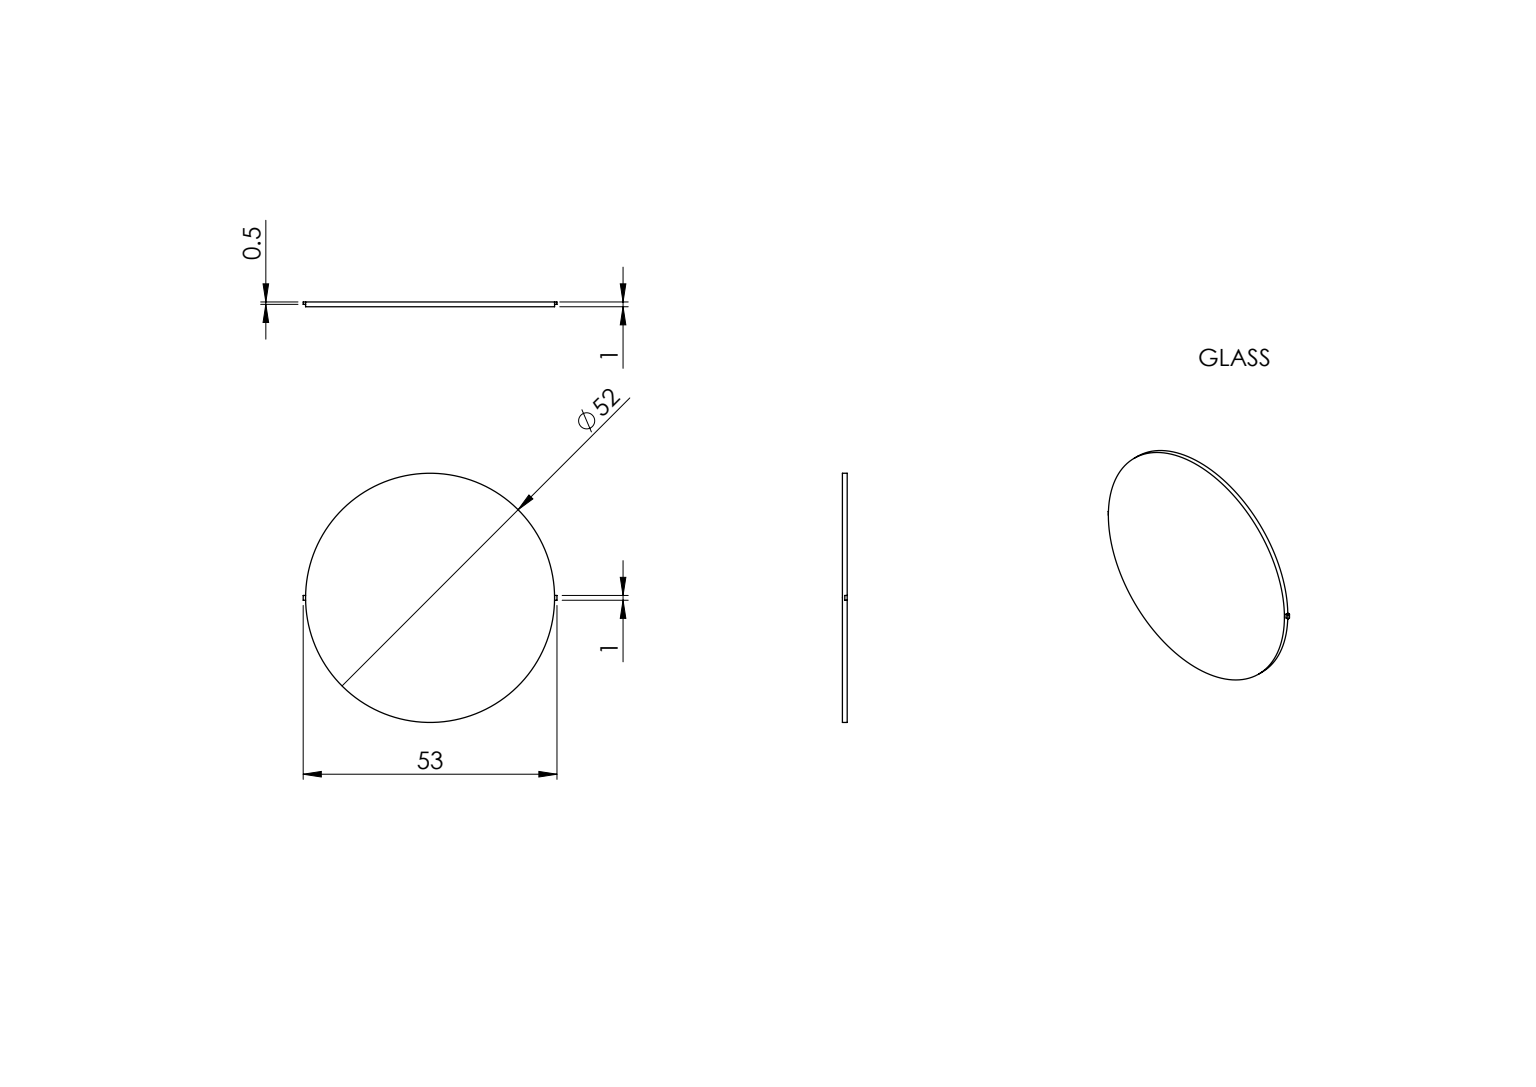
ISO-10303-21;
HEADER;
FILE_DESCRIPTION (('STEP AP214'),
    '1' );
FILE_NAME ('glass.step',
    '2026-10-26T11:20:31',
    ( '' ),
    ( '' ),
    'SwSTEP 2.0',
    'SolidWorks 2026',
    '' );
FILE_SCHEMA (( 'AUTOMOTIVE_DESIGN' ));
ENDSEC;

DATA;
#34=ORIENTED_EDGE ( 'NONE', *, *, #3765, .T. ) ;
#67=FACE_OUTER_BOUND ( 'NONE', #3163, .T. ) ;
#75=ORIENTED_EDGE ( 'NONE', *, *, #1897, .F. ) ;
#83=PLANE ( 'NONE',  #429 ) ;
#102=VERTEX_POINT ( 'NONE', #652 ) ;
#124=ORIENTED_EDGE ( 'NONE', *, *, #3765, .F. ) ;
#132=EDGE_CURVE ( 'NONE', #2734, #2850, #1760, .T. ) ;
#136=AXIS2_PLACEMENT_3D ( 'NONE', #3423, #167, #2705 ) ;
#142=EDGE_CURVE ( 'NONE', #3182, #1602, #2491, .T. ) ;
#147=CARTESIAN_POINT ( 'NONE',  ( 0.000000000000000000, 0.000000000000000000, 20.00000000000000000 ) ) ;
#167=DIRECTION ( 'NONE',  ( 0.000000000000000000, -0.000000000000000000, 1.000000000000000000 ) ) ;
#206=PRODUCT ( 'glass', 'glass', '', ( #2572 ) ) ;
#214=ORIENTED_EDGE ( 'NONE', *, *, #364, .F. ) ;
#229=EDGE_CURVE ( 'NONE', #3297, #3886, #3090, .T. ) ;
#234=CARTESIAN_POINT ( 'NONE',  ( 26.49999999999999645, -0.5000000000000000000, 19.50000000000000000 ) ) ;
#248=VECTOR ( 'NONE', #2476, 1000.000000000000000 ) ;
#285=LINE ( 'NONE', #1756, #509 ) ;
#331=PLANE ( 'NONE',  #3572 ) ;
#364=EDGE_CURVE ( 'NONE', #2850, #4511, #2465, .T. ) ;
#369=DIRECTION ( 'NONE',  ( -1.000000000000000000, 0.000000000000000000, 0.000000000000000000 ) ) ;
#389=CARTESIAN_POINT ( 'NONE',  ( 26.00000000000000711, 3.184081677783118980E-15, 20.00000000000000000 ) ) ;
#398=FACE_OUTER_BOUND ( 'NONE', #695, .T. ) ;
#413=VECTOR ( 'NONE', #4600, 1000.000000000000000 ) ;
#418=VERTEX_POINT ( 'NONE', #4346 ) ;
#422=APPLICATION_CONTEXT ( 'automotive_design' ) ;
#425=ADVANCED_FACE ( 'NONE', ( #2551 ), #3201, .T. ) ;
#426=ORIENTED_EDGE ( 'NONE', *, *, #1762, .F. ) ;
#429=AXIS2_PLACEMENT_3D ( 'NONE', #1371, #641, #2955 ) ;
#437=AXIS2_PLACEMENT_3D ( 'NONE', #3171, #2146, #3524 ) ;
#440=VECTOR ( 'NONE', #3448, 1000.000000000000000 ) ;
#456=VECTOR ( 'NONE', #3934, 1000.000000000000000 ) ;
#463=VECTOR ( 'NONE', #1245, 1000.000000000000000 ) ;
#483=ORIENTED_EDGE ( 'NONE', *, *, #4706, .T. ) ;
#488=CIRCLE ( 'NONE', #2609, 26.00000000000000711 ) ;
#492=ORIENTED_EDGE ( 'NONE', *, *, #132, .T. ) ;
#509=VECTOR ( 'NONE', #2115, 1000.000000000000000 ) ;
#517=CARTESIAN_POINT ( 'NONE',  ( 26.49999999999999645, 0.5000000000000000000, 19.00000000000000000 ) ) ;
#552=LINE ( 'NONE', #1733, #440 ) ;
#572=ORIENTED_EDGE ( 'NONE', *, *, #4588, .T. ) ;
#612=CARTESIAN_POINT ( 'NONE',  ( -25.99519186311192342, -0.5000000000000000000, 19.50000000000000000 ) ) ;
#620=ADVANCED_FACE ( 'NONE', ( #67 ), #1945, .T. ) ;
#625=CARTESIAN_POINT ( 'NONE',  ( 25.99519186311192342, -0.5000000000000000000, 19.50000000000000000 ) ) ;
#627=( NAMED_UNIT ( * ) SI_UNIT ( $, .STERADIAN. ) SOLID_ANGLE_UNIT ( ) );
#633=CARTESIAN_POINT ( 'NONE',  ( 26.49999999999999645, 0.5000000000000000000, 19.00000000000000000 ) ) ;
#641=DIRECTION ( 'NONE',  ( -1.000000000000000000, 0.000000000000000000, 0.000000000000000000 ) ) ;
#645=ORIENTED_EDGE ( 'NONE', *, *, #2272, .F. ) ;
#652=CARTESIAN_POINT ( 'NONE',  ( 26.49999999999999645, 0.5000000000000000000, 19.50000000000000000 ) ) ;
#672=FILL_AREA_STYLE ('',( #2807 ) ) ;
#676=DIRECTION ( 'NONE',  ( 1.000000000000000000, 0.000000000000000000, 0.000000000000000000 ) ) ;
#682=AXIS2_PLACEMENT_3D ( 'NONE', #4584, #4229, #972 ) ;
#695=EDGE_LOOP ( 'NONE', ( #214, #1153, #2156, #1634, #75 ) ) ;
#754=STYLED_ITEM('',(#4729),#2889);
#777=EDGE_CURVE ( 'NONE', #1588, #3297, #4191, .T. ) ;
#824=VECTOR ( 'NONE', #4005, 1000.000000000000000 ) ;
#827=ORIENTED_EDGE ( 'NONE', *, *, #3495, .T. ) ;
#835=ORIENTED_EDGE ( 'NONE', *, *, #777, .T. ) ;
#839=PRODUCT_DEFINITION ( 'UNKNOWN', '', #2243, #1713 ) ;
#856=ORIENTED_EDGE ( 'NONE', *, *, #4405, .T. ) ;
#863=EDGE_CURVE ( 'NONE', #4361, #4498, #4302, .T. ) ;
#888=DIRECTION ( 'NONE',  ( 1.000000000000000000, -0.000000000000000000, -0.000000000000000000 ) ) ;
#896=ADVANCED_FACE ( 'NONE', ( #1497 ), #83, .T. ) ;
#901=CARTESIAN_POINT ( 'NONE',  ( 0.000000000000000000, 0.000000000000000000, 19.50000000000000000 ) ) ;
#931=EDGE_LOOP ( 'NONE', ( #3447, #2373, #34, #4420, #3973, #4198, #492, #4425 ) ) ;
#935=ORIENTED_EDGE ( 'NONE', *, *, #2783, .T. ) ;
#960=ADVANCED_FACE ( 'NONE', ( #4674 ), #2853, .T. ) ;
#972=DIRECTION ( 'NONE',  ( 1.000000000000000000, 0.000000000000000000, 0.000000000000000000 ) ) ;
#981=ORIENTED_EDGE ( 'NONE', *, *, #1897, .T. ) ;
#983=LINE ( 'NONE', #4201, #2873 ) ;
#996=LINE ( 'NONE', #2062, #248 ) ;
#998=CARTESIAN_POINT ( 'NONE',  ( 26.49999999999999645, -0.5000000000000000000, 19.00000000000000000 ) ) ;
#1003=PRESENTATION_STYLE_ASSIGNMENT (( #2485 ) ) ;
#1010=ORIENTED_EDGE ( 'NONE', *, *, #142, .F. ) ;
#1029=CARTESIAN_POINT ( 'NONE',  ( 25.99519186311192342, -0.5000000000000000000, 20.00000000000000000 ) ) ;
#1037=COLOUR_RGB ( '',0.8941176470588234615, 0.8941176470588234615, 0.8941176470588234615 ) ;
#1039=CARTESIAN_POINT ( 'NONE',  ( -26.50000000000000355, 0.5000000000000000000, 19.50000000000000000 ) ) ;
#1045=CARTESIAN_POINT ( 'NONE',  ( 0.000000000000000000, 0.000000000000000000, 20.00000000000000000 ) ) ;
#1091=ADVANCED_FACE ( 'NONE', ( #398 ), #331, .T. ) ;
#1113=DIRECTION ( 'NONE',  ( 1.000000000000000000, 0.000000000000000000, 0.000000000000000000 ) ) ;
#1114=CYLINDRICAL_SURFACE ( 'NONE', #4514, 26.00000000000000711 ) ;
#1115=DIRECTION ( 'NONE',  ( 0.000000000000000000, 0.000000000000000000, -1.000000000000000000 ) ) ;
#1131=EDGE_CURVE ( 'NONE', #3723, #2120, #2345, .T. ) ;
#1138=CARTESIAN_POINT ( 'NONE',  ( 0.000000000000000000, 0.000000000000000000, 19.00000000000000000 ) ) ;
#1153=ORIENTED_EDGE ( 'NONE', *, *, #2783, .F. ) ;
#1184=( GEOMETRIC_REPRESENTATION_CONTEXT ( 3 ) GLOBAL_UNCERTAINTY_ASSIGNED_CONTEXT ( ( #1246 ) ) GLOBAL_UNIT_ASSIGNED_CONTEXT ( ( #1619, #2368, #2391 ) ) REPRESENTATION_CONTEXT ( 'NONE', 'WORKASPACE' ) );
#1218=ORIENTED_EDGE ( 'NONE', *, *, #4706, .F. ) ;
#1236=VECTOR ( 'NONE', #2396, 1000.000000000000000 ) ;
#1245=DIRECTION ( 'NONE',  ( 1.000000000000000000, -0.000000000000000000, -0.000000000000000000 ) ) ;
#1246=UNCERTAINTY_MEASURE_WITH_UNIT (LENGTH_MEASURE( 1.000000000000000082E-05 ), #1619, 'distance_accuracy_value', 'NONE');
#1249=EDGE_CURVE ( 'NONE', #3723, #4511, #4529, .T. ) ;
#1250=EDGE_CURVE ( 'NONE', #418, #102, #3047, .T. ) ;
#1289=ORIENTED_EDGE ( 'NONE', *, *, #4086, .T. ) ;
#1310=CARTESIAN_POINT ( 'NONE',  ( 0.000000000000000000, 0.000000000000000000, 19.50000000000000000 ) ) ;
#1332=CARTESIAN_POINT ( 'NONE',  ( 26.49999999999999645, -0.5000000000000000000, 19.50000000000000000 ) ) ;
#1346=CARTESIAN_POINT ( 'NONE',  ( 25.99519186311192342, 0.5000000000000000000, 20.00000000000000000 ) ) ;
#1350=ORIENTED_EDGE ( 'NONE', *, *, #4588, .F. ) ;
#1361=ADVANCED_FACE ( 'NONE', ( #3429 ), #3142, .F. ) ;
#1366=CARTESIAN_POINT ( 'NONE',  ( 26.49999999999999645, -0.5000000000000000000, 19.50000000000000000 ) ) ;
#1371=CARTESIAN_POINT ( 'NONE',  ( -26.50000000000000355, -0.5000000000000000000, 19.50000000000000000 ) ) ;
#1398=ORIENTED_EDGE ( 'NONE', *, *, #2495, .F. ) ;
#1410=LINE ( 'NONE', #1366, #2230 ) ;
#1419=CARTESIAN_POINT ( 'NONE',  ( -26.50000000000000355, -0.5000000000000000000, 19.50000000000000000 ) ) ;
#1428=AXIS2_PLACEMENT_3D ( 'NONE', #3216, #2419, #4656 ) ;
#1442=AXIS2_PLACEMENT_3D ( 'NONE', #901, #3806, #1607 ) ;
#1449=EDGE_LOOP ( 'NONE', ( #1010, #1696, #3014, #3137, #2336 ) ) ;
#1497=FACE_OUTER_BOUND ( 'NONE', #2181, .T. ) ;
#1501=CARTESIAN_POINT ( 'NONE',  ( 26.49999999999999645, 0.5000000000000000000, 19.50000000000000000 ) ) ;
#1521=CARTESIAN_POINT ( 'NONE',  ( 26.00000000000000711, 3.184081677783118980E-15, 19.50000000000000000 ) ) ;
#1529=CIRCLE ( 'NONE', #2070, 26.00000000000000711 ) ;
#1537=DIRECTION ( 'NONE',  ( 1.000000000000000000, 0.000000000000000000, 0.000000000000000000 ) ) ;
#1542=ORIENTED_EDGE ( 'NONE', *, *, #1131, .T. ) ;
#1548=EDGE_CURVE ( 'NONE', #1588, #3303, #2283, .T. ) ;
#1588=VERTEX_POINT ( 'NONE', #3015 ) ;
#1591=ORIENTED_EDGE ( 'NONE', *, *, #142, .T. ) ;
#1602=VERTEX_POINT ( 'NONE', #3440 ) ;
#1607=DIRECTION ( 'NONE',  ( 1.000000000000000000, 0.000000000000000000, 0.000000000000000000 ) ) ;
#1619=( LENGTH_UNIT ( ) NAMED_UNIT ( * ) SI_UNIT ( .MILLI., .METRE. ) );
#1626=ORIENTED_EDGE ( 'NONE', *, *, #1131, .F. ) ;
#1634=ORIENTED_EDGE ( 'NONE', *, *, #1250, .F. ) ;
#1639=MECHANICAL_DESIGN_GEOMETRIC_PRESENTATION_REPRESENTATION('',(#4159),#4692);
#1647=EDGE_CURVE ( 'NONE', #1602, #4361, #4265, .T. ) ;
#1653=DIRECTION ( 'NONE',  ( 1.000000000000000000, -0.000000000000000000, -0.000000000000000000 ) ) ;
#1662=VECTOR ( 'NONE', #3899, 1000.000000000000000 ) ;
#1667=ORIENTED_EDGE ( 'NONE', *, *, #777, .F. ) ;
#1696=ORIENTED_EDGE ( 'NONE', *, *, #4086, .F. ) ;
#1712=DIRECTION ( 'NONE',  ( 0.000000000000000000, 0.000000000000000000, 1.000000000000000000 ) ) ;
#1713=PRODUCT_DEFINITION_CONTEXT ( 'detailed design', #3498, 'design' ) ;
#1730=ORIENTED_EDGE ( 'NONE', *, *, #2329, .T. ) ;
#1733=CARTESIAN_POINT ( 'NONE',  ( 26.49999999999999645, -0.5000000000000000000, 19.50000000000000000 ) ) ;
#1736=SURFACE_STYLE_FILL_AREA ( #672 ) ;
#1741=CARTESIAN_POINT ( 'NONE',  ( -25.99519186311192342, 0.5000000000000000000, 19.50000000000000000 ) ) ;
#1755=ORIENTED_EDGE ( 'NONE', *, *, #2918, .T. ) ;
#1756=CARTESIAN_POINT ( 'NONE',  ( 26.49999999999999645, 0.5000000000000000000, 19.50000000000000000 ) ) ;
#1759=VERTEX_POINT ( 'NONE', #1332 ) ;
#1760=LINE ( 'NONE', #1029, #456 ) ;
#1762=EDGE_CURVE ( 'NONE', #2297, #2553, #996, .T. ) ;
#1765=PLANE ( 'NONE',  #1428 ) ;
#1773=CARTESIAN_POINT ( 'NONE',  ( 26.49999999999999645, -0.5000000000000000000, 19.50000000000000000 ) ) ;
#1775=ORIENTED_EDGE ( 'NONE', *, *, #1250, .T. ) ;
#1780=CARTESIAN_POINT ( 'NONE',  ( 0.000000000000000000, 0.000000000000000000, 0.000000000000000000 ) ) ;
#1788=ADVANCED_FACE ( 'NONE', ( #2867 ), #4689, .T. ) ;
#1817=DIRECTION ( 'NONE',  ( 0.000000000000000000, -0.000000000000000000, 1.000000000000000000 ) ) ;
#1837=AXIS2_PLACEMENT_3D ( 'NONE', #3841, #2834, #3170 ) ;
#1893=VECTOR ( 'NONE', #2752, 1000.000000000000000 ) ;
#1895=ORIENTED_EDGE ( 'NONE', *, *, #229, .F. ) ;
#1897=EDGE_CURVE ( 'NONE', #4511, #418, #1529, .T. ) ;
#1904=ORIENTED_EDGE ( 'NONE', *, *, #1548, .F. ) ;
#1907=AXIS2_PLACEMENT_3D ( 'NONE', #147, #2315, #1953 ) ;
#1920=CARTESIAN_POINT ( 'NONE',  ( -26.00000000000000711, 0.000000000000000000, 20.00000000000000000 ) ) ;
#1939=LINE ( 'NONE', #1501, #3753 ) ;
#1945=PLANE ( 'NONE',  #3771 ) ;
#1953=DIRECTION ( 'NONE',  ( 1.000000000000000000, 0.000000000000000000, 0.000000000000000000 ) ) ;
#1987=ORIENTED_EDGE ( 'NONE', *, *, #2862, .F. ) ;
#2003=DIRECTION ( 'NONE',  ( 1.000000000000000000, 0.000000000000000000, -0.000000000000000000 ) ) ;
#2042=PLANE ( 'NONE',  #2947 ) ;
#2047=CIRCLE ( 'NONE', #682, 26.00000000000000711 ) ;
#2062=CARTESIAN_POINT ( 'NONE',  ( -26.50000000000000355, -0.5000000000000000000, 19.00000000000000000 ) ) ;
#2070=AXIS2_PLACEMENT_3D ( 'NONE', #2174, #1817, #1113 ) ;
#2074=DIRECTION ( 'NONE',  ( -1.000000000000000000, 0.000000000000000000, 0.000000000000000000 ) ) ;
#2099=FACE_OUTER_BOUND ( 'NONE', #3630, .T. ) ;
#2105=DIRECTION ( 'NONE',  ( -0.000000000000000000, -0.000000000000000000, -1.000000000000000000 ) ) ;
#2115=DIRECTION ( 'NONE',  ( 0.000000000000000000, 0.000000000000000000, -1.000000000000000000 ) ) ;
#2120=VERTEX_POINT ( 'NONE', #3716 ) ;
#2122=FACE_OUTER_BOUND ( 'NONE', #931, .T. ) ;
#2146=DIRECTION ( 'NONE',  ( 0.000000000000000000, 0.000000000000000000, 1.000000000000000000 ) ) ;
#2149=DIRECTION ( 'NONE',  ( 0.000000000000000000, 0.000000000000000000, -1.000000000000000000 ) ) ;
#2151=DIRECTION ( 'NONE',  ( 0.000000000000000000, 0.000000000000000000, -1.000000000000000000 ) ) ;
#2156=ORIENTED_EDGE ( 'NONE', *, *, #2755, .F. ) ;
#2174=CARTESIAN_POINT ( 'NONE',  ( 0.000000000000000000, 0.000000000000000000, 19.50000000000000000 ) ) ;
#2176=DIRECTION ( 'NONE',  ( 0.000000000000000000, -1.000000000000000000, -0.000000000000000000 ) ) ;
#2181=EDGE_LOOP ( 'NONE', ( #426, #3756, #3738, #4433 ) ) ;
#2230=VECTOR ( 'NONE', #3172, 1000.000000000000000 ) ;
#2243=PRODUCT_DEFINITION_FORMATION_WITH_SPECIFIED_SOURCE ( 'ANY', '', #206, .NOT_KNOWN. ) ;
#2272=EDGE_CURVE ( 'NONE', #418, #1588, #4245, .T. ) ;
#2280=ADVANCED_FACE ( 'NONE', ( #2122 ), #3545, .T. ) ;
#2283=CIRCLE ( 'NONE', #3355, 26.00000000000000711 ) ;
#2297=VERTEX_POINT ( 'NONE', #3935 ) ;
#2299=CARTESIAN_POINT ( 'NONE',  ( 0.000000000000000000, 0.000000000000000000, 19.00000000000000000 ) ) ;
#2315=DIRECTION ( 'NONE',  ( 0.000000000000000000, 0.000000000000000000, 1.000000000000000000 ) ) ;
#2321=DIRECTION ( 'NONE',  ( 0.000000000000000000, 0.000000000000000000, 1.000000000000000000 ) ) ;
#2326=ORIENTED_EDGE ( 'NONE', *, *, #3794, .F. ) ;
#2329=EDGE_CURVE ( 'NONE', #4361, #2996, #3864, .T. ) ;
#2336=ORIENTED_EDGE ( 'NONE', *, *, #1647, .F. ) ;
#2345=CIRCLE ( 'NONE', #1907, 26.00000000000000711 ) ;
#2368=( NAMED_UNIT ( * ) PLANE_ANGLE_UNIT ( ) SI_UNIT ( $, .RADIAN. ) );
#2373=ORIENTED_EDGE ( 'NONE', *, *, #2918, .F. ) ;
#2391=( NAMED_UNIT ( * ) SI_UNIT ( $, .STERADIAN. ) SOLID_ANGLE_UNIT ( ) );
#2396=DIRECTION ( 'NONE',  ( -0.000000000000000000, -0.000000000000000000, -1.000000000000000000 ) ) ;
#2407=LINE ( 'NONE', #4568, #1893 ) ;
#2415=LINE ( 'NONE', #2461, #413 ) ;
#2417=DIRECTION ( 'NONE',  ( 0.000000000000000000, -0.000000000000000000, 1.000000000000000000 ) ) ;
#2419=DIRECTION ( 'NONE',  ( 0.000000000000000000, 1.000000000000000000, 0.000000000000000000 ) ) ;
#2461=CARTESIAN_POINT ( 'NONE',  ( 26.49999999999999645, -0.5000000000000000000, 19.00000000000000000 ) ) ;
#2465=CIRCLE ( 'NONE', #136, 26.00000000000000711 ) ;
#2471=( NAMED_UNIT ( * ) SI_UNIT ( $, .STERADIAN. ) SOLID_ANGLE_UNIT ( ) );
#2476=DIRECTION ( 'NONE',  ( 0.000000000000000000, 1.000000000000000000, 0.000000000000000000 ) ) ;
#2485=SURFACE_STYLE_USAGE ( .BOTH. , #4264 ) ;
#2491=CIRCLE ( 'NONE', #3364, 26.00000000000000711 ) ;
#2495=EDGE_CURVE ( 'NONE', #3886, #2734, #4380, .T. ) ;
#2501=VECTOR ( 'NONE', #2759, 1000.000000000000000 ) ;
#2511=DIRECTION ( 'NONE',  ( 0.000000000000000000, -0.000000000000000000, 1.000000000000000000 ) ) ;
#2536=CARTESIAN_POINT ( 'NONE',  ( 26.49999999999999645, -0.5000000000000000000, 19.00000000000000000 ) ) ;
#2551=FACE_OUTER_BOUND ( 'NONE', #3658, .T. ) ;
#2553=VERTEX_POINT ( 'NONE', #4428 ) ;
#2572=PRODUCT_CONTEXT ( 'NONE', #422, 'mechanical' ) ;
#2575=DIRECTION ( 'NONE',  ( 1.000000000000000000, 0.000000000000000000, 0.000000000000000000 ) ) ;
#2609=AXIS2_PLACEMENT_3D ( 'NONE', #1138, #3777, #2575 ) ;
#2614=VECTOR ( 'NONE', #2149, 1000.000000000000000 ) ;
#2658=ORIENTED_EDGE ( 'NONE', *, *, #2755, .T. ) ;
#2662=UNCERTAINTY_MEASURE_WITH_UNIT (LENGTH_MEASURE( 1.000000000000000082E-05 ), #2852, 'distance_accuracy_value', 'NONE');
#2673=VECTOR ( 'NONE', #4518, 1000.000000000000000 ) ;
#2685=LINE ( 'NONE', #4152, #4149 ) ;
#2705=DIRECTION ( 'NONE',  ( 1.000000000000000000, 0.000000000000000000, 0.000000000000000000 ) ) ;
#2720=ORIENTED_EDGE ( 'NONE', *, *, #2862, .T. ) ;
#2734=VERTEX_POINT ( 'NONE', #3859 ) ;
#2736=CARTESIAN_POINT ( 'NONE',  ( 26.00000000000000711, 3.184081677783118980E-15, 20.00000000000000000 ) ) ;
#2752=DIRECTION ( 'NONE',  ( 0.000000000000000000, 0.000000000000000000, -1.000000000000000000 ) ) ;
#2754=ORIENTED_EDGE ( 'NONE', *, *, #2495, .T. ) ;
#2755=EDGE_CURVE ( 'NONE', #102, #1759, #552, .T. ) ;
#2759=DIRECTION ( 'NONE',  ( -0.000000000000000000, -0.000000000000000000, -1.000000000000000000 ) ) ;
#2778=VECTOR ( 'NONE', #1653, 1000.000000000000000 ) ;
#2783=EDGE_CURVE ( 'NONE', #1759, #2850, #983, .T. ) ;
#2807=FILL_AREA_STYLE_COLOUR ( '', #1037 ) ;
#2812=CARTESIAN_POINT ( 'NONE',  ( 26.49999999999999645, -0.5000000000000000000, 19.50000000000000000 ) ) ;
#2834=DIRECTION ( 'NONE',  ( -0.000000000000000000, -0.000000000000000000, -1.000000000000000000 ) ) ;
#2839=EDGE_CURVE ( 'NONE', #3303, #3182, #3120, .T. ) ;
#2850=VERTEX_POINT ( 'NONE', #625 ) ;
#2852=( LENGTH_UNIT ( ) NAMED_UNIT ( * ) SI_UNIT ( .MILLI., .METRE. ) );
#2853=PLANE ( 'NONE',  #3692 ) ;
#2862=EDGE_CURVE ( 'NONE', #102, #3297, #285, .T. ) ;
#2867=FACE_OUTER_BOUND ( 'NONE', #4572, .T. ) ;
#2873=VECTOR ( 'NONE', #4596, 1000.000000000000000 ) ;
#2876=DIRECTION ( 'NONE',  ( 0.000000000000000000, 0.000000000000000000, -1.000000000000000000 ) ) ;
#2889=MANIFOLD_SOLID_BREP ( 'Boss-Extrude2', #3434 ) ;
#2891=LINE ( 'NONE', #1419, #3373 ) ;
#2900=CARTESIAN_POINT ( 'NONE',  ( 26.49999999999999645, -0.5000000000000000000, 19.50000000000000000 ) ) ;
#2918=EDGE_CURVE ( 'NONE', #2120, #3723, #2047, .T. ) ;
#2928=AXIS2_PLACEMENT_3D ( 'NONE', #1780, #1712, #3957 ) ;
#2945=ORIENTED_EDGE ( 'NONE', *, *, #2839, .T. ) ;
#2947=AXIS2_PLACEMENT_3D ( 'NONE', #1310, #4256, #3852 ) ;
#2955=DIRECTION ( 'NONE',  ( 0.000000000000000000, 0.000000000000000000, 1.000000000000000000 ) ) ;
#2963=DIRECTION ( 'NONE',  ( -0.000000000000000000, -0.000000000000000000, -1.000000000000000000 ) ) ;
#2996=VERTEX_POINT ( 'NONE', #3337 ) ;
#3012=DIRECTION ( 'NONE',  ( 0.000000000000000000, 1.000000000000000000, 0.000000000000000000 ) ) ;
#3014=ORIENTED_EDGE ( 'NONE', *, *, #3698, .F. ) ;
#3015=CARTESIAN_POINT ( 'NONE',  ( 25.99519186311192342, 0.5000000000000000000, 19.00000000000000000 ) ) ;
#3016=CARTESIAN_POINT ( 'NONE',  ( -25.99519186311192342, 0.5000000000000000000, 19.00000000000000000 ) ) ;
#3030=DIRECTION ( 'NONE',  ( 1.000000000000000000, -0.000000000000000000, -0.000000000000000000 ) ) ;
#3047=LINE ( 'NONE', #4575, #463 ) ;
#3050=SHAPE_REPRESENTATION ( 'glass', ( #2928 ), #1184 ) ;
#3090=LINE ( 'NONE', #998, #2673 ) ;
#3120=LINE ( 'NONE', #3878, #1662 ) ;
#3128=AXIS2_PLACEMENT_3D ( 'NONE', #2299, #2321, #2003 ) ;
#3134=DIRECTION ( 'NONE',  ( 1.000000000000000000, -0.000000000000000000, 0.000000000000000000 ) ) ;
#3137=ORIENTED_EDGE ( 'NONE', *, *, #2329, .F. ) ;
#3142=PLANE ( 'NONE',  #3128 ) ;
#3163=EDGE_LOOP ( 'NONE', ( #3260, #1350, #4144, #1289 ) ) ;
#3170=DIRECTION ( 'NONE',  ( -1.000000000000000000, 0.000000000000000000, 0.000000000000000000 ) ) ;
#3171=CARTESIAN_POINT ( 'NONE',  ( 0.000000000000000000, 0.000000000000000000, 20.00000000000000000 ) ) ;
#3172=DIRECTION ( 'NONE',  ( 0.000000000000000000, 0.000000000000000000, -1.000000000000000000 ) ) ;
#3174=LINE ( 'NONE', #3196, #2614 ) ;
#3182=VERTEX_POINT ( 'NONE', #1741 ) ;
#3187=( NAMED_UNIT ( * ) PLANE_ANGLE_UNIT ( ) SI_UNIT ( $, .RADIAN. ) );
#3195=( LENGTH_UNIT ( ) NAMED_UNIT ( * ) SI_UNIT ( .MILLI., .METRE. ) );
#3196=CARTESIAN_POINT ( 'NONE',  ( -26.50000000000000355, 0.5000000000000000000, 19.50000000000000000 ) ) ;
#3201=PLANE ( 'NONE',  #3236 ) ;
#3211=ADVANCED_FACE ( 'NONE', ( #4246 ), #4337, .T. ) ;
#3212=ORIENTED_EDGE ( 'NONE', *, *, #229, .T. ) ;
#3216=CARTESIAN_POINT ( 'NONE',  ( 26.49999999999999645, 0.5000000000000000000, 19.50000000000000000 ) ) ;
#3236=AXIS2_PLACEMENT_3D ( 'NONE', #1773, #2176, #1115 ) ;
#3242=ADVANCED_FACE ( 'NONE', ( #2099 ), #1765, .T. ) ;
#3248=FACE_OUTER_BOUND ( 'NONE', #4333, .T. ) ;
#3254=MECHANICAL_DESIGN_GEOMETRIC_PRESENTATION_REPRESENTATION('',(#754),#3331);
#3260=ORIENTED_EDGE ( 'NONE', *, *, #2839, .F. ) ;
#3297=VERTEX_POINT ( 'NONE', #633 ) ;
#3303=VERTEX_POINT ( 'NONE', #3016 ) ;
#3321=DIRECTION ( 'NONE',  ( 0.000000000000000000, 0.000000000000000000, 1.000000000000000000 ) ) ;
#3331=( GEOMETRIC_REPRESENTATION_CONTEXT ( 3 ) GLOBAL_UNCERTAINTY_ASSIGNED_CONTEXT ( ( #3354 ) ) GLOBAL_UNIT_ASSIGNED_CONTEXT ( ( #3195, #3485, #2471 ) ) REPRESENTATION_CONTEXT ( 'NONE', 'WORKASPACE' ) );
#3337=CARTESIAN_POINT ( 'NONE',  ( -26.50000000000000355, -0.5000000000000000000, 19.50000000000000000 ) ) ;
#3354=UNCERTAINTY_MEASURE_WITH_UNIT (LENGTH_MEASURE( 1.000000000000000082E-05 ), #3195, 'distance_accuracy_value', 'NONE');
#3355=AXIS2_PLACEMENT_3D ( 'NONE', #3701, #3321, #1537 ) ;
#3364=AXIS2_PLACEMENT_3D ( 'NONE', #3568, #2417, #676 ) ;
#3373=VECTOR ( 'NONE', #4324, 1000.000000000000000 ) ;
#3423=CARTESIAN_POINT ( 'NONE',  ( 0.000000000000000000, 0.000000000000000000, 19.50000000000000000 ) ) ;
#3429=FACE_OUTER_BOUND ( 'NONE', #4543, .T. ) ;
#3434=CLOSED_SHELL ( 'NONE', ( #3633, #2280, #3211, #1361, #1788, #1091, #3242, #960, #3452, #425, #620, #896 ) ) ;
#3440=CARTESIAN_POINT ( 'NONE',  ( -26.00000000000000711, 0.000000000000000000, 19.50000000000000000 ) ) ;
#3447=ORIENTED_EDGE ( 'NONE', *, *, #1249, .F. ) ;
#3448=DIRECTION ( 'NONE',  ( -0.000000000000000000, -1.000000000000000000, -0.000000000000000000 ) ) ;
#3452=ADVANCED_FACE ( 'NONE', ( #3807 ), #2042, .T. ) ;
#3485=( NAMED_UNIT ( * ) PLANE_ANGLE_UNIT ( ) SI_UNIT ( $, .RADIAN. ) );
#3495=EDGE_CURVE ( 'NONE', #2996, #2297, #2407, .T. ) ;
#3498=APPLICATION_CONTEXT ( 'automotive_design' ) ;
#3505=PRODUCT_DEFINITION_SHAPE ( 'NONE', 'NONE',  #839 ) ;
#3524=DIRECTION ( 'NONE',  ( 1.000000000000000000, 0.000000000000000000, -0.000000000000000000 ) ) ;
#3545=CYLINDRICAL_SURFACE ( 'NONE', #1837, 26.00000000000000711 ) ;
#3568=CARTESIAN_POINT ( 'NONE',  ( 0.000000000000000000, 0.000000000000000000, 19.50000000000000000 ) ) ;
#3572=AXIS2_PLACEMENT_3D ( 'NONE', #4699, #2511, #3977 ) ;
#3575=SHAPE_DEFINITION_REPRESENTATION ( #3505, #3050 ) ;
#3586=VECTOR ( 'NONE', #2074, 1000.000000000000000 ) ;
#3588=SHAPE_REPRESENTATION_RELATIONSHIP ( 'NONE' , 'NONE' ,  #3050, #3930 ) ;
#3630=EDGE_LOOP ( 'NONE', ( #645, #1775, #2720, #1667 ) ) ;
#3633=ADVANCED_FACE ( 'NONE', ( #3248 ), #1114, .T. ) ;
#3639=ORIENTED_EDGE ( 'NONE', *, *, #2272, .T. ) ;
#3643=ORIENTED_EDGE ( 'NONE', *, *, #4405, .F. ) ;
#3650=DIRECTION ( 'NONE',  ( -0.000000000000000000, -0.000000000000000000, -1.000000000000000000 ) ) ;
#3658=EDGE_LOOP ( 'NONE', ( #4048, #1730, #827, #1218 ) ) ;
#3692=AXIS2_PLACEMENT_3D ( 'NONE', #2900, #4354, #2876 ) ;
#3698=EDGE_CURVE ( 'NONE', #2996, #3949, #2891, .T. ) ;
#3701=CARTESIAN_POINT ( 'NONE',  ( 0.000000000000000000, 0.000000000000000000, 19.00000000000000000 ) ) ;
#3716=CARTESIAN_POINT ( 'NONE',  ( -26.00000000000000711, 0.000000000000000000, 20.00000000000000000 ) ) ;
#3720=LINE ( 'NONE', #1920, #4362 ) ;
#3723=VERTEX_POINT ( 'NONE', #389 ) ;
#3738=ORIENTED_EDGE ( 'NONE', *, *, #3698, .T. ) ;
#3753=VECTOR ( 'NONE', #3030, 1000.000000000000000 ) ;
#3756=ORIENTED_EDGE ( 'NONE', *, *, #3495, .F. ) ;
#3765=EDGE_CURVE ( 'NONE', #2120, #1602, #3720, .T. ) ;
#3771=AXIS2_PLACEMENT_3D ( 'NONE', #4491, #3012, #4467 ) ;
#3777=DIRECTION ( 'NONE',  ( 0.000000000000000000, 0.000000000000000000, 1.000000000000000000 ) ) ;
#3784=ORIENTED_EDGE ( 'NONE', *, *, #132, .F. ) ;
#3794=EDGE_CURVE ( 'NONE', #4498, #2734, #488, .T. ) ;
#3806=DIRECTION ( 'NONE',  ( 0.000000000000000000, -0.000000000000000000, 1.000000000000000000 ) ) ;
#3807=FACE_OUTER_BOUND ( 'NONE', #1449, .T. ) ;
#3841=CARTESIAN_POINT ( 'NONE',  ( 0.000000000000000000, 0.000000000000000000, 20.00000000000000000 ) ) ;
#3852=DIRECTION ( 'NONE',  ( 1.000000000000000000, 0.000000000000000000, -0.000000000000000000 ) ) ;
#3859=CARTESIAN_POINT ( 'NONE',  ( 25.99519186311192342, -0.5000000000000000000, 19.00000000000000000 ) ) ;
#3864=LINE ( 'NONE', #2812, #3586 ) ;
#3878=CARTESIAN_POINT ( 'NONE',  ( -25.99519186311192342, 0.5000000000000000000, 20.00000000000000000 ) ) ;
#3886=VERTEX_POINT ( 'NONE', #3892 ) ;
#3892=CARTESIAN_POINT ( 'NONE',  ( 26.49999999999999645, -0.5000000000000000000, 19.00000000000000000 ) ) ;
#3899=DIRECTION ( 'NONE',  ( 0.000000000000000000, 0.000000000000000000, 1.000000000000000000 ) ) ;
#3929=VECTOR ( 'NONE', #2105, 1000.000000000000000 ) ;
#3930=ADVANCED_BREP_SHAPE_REPRESENTATION ( '', ( #2889, #2928 ), #1184 ) ;
#3934=DIRECTION ( 'NONE',  ( 0.000000000000000000, 0.000000000000000000, 1.000000000000000000 ) ) ;
#3935=CARTESIAN_POINT ( 'NONE',  ( -26.50000000000000355, -0.5000000000000000000, 19.00000000000000000 ) ) ;
#3949=VERTEX_POINT ( 'NONE', #1039 ) ;
#3957=DIRECTION ( 'NONE',  ( 1.000000000000000000, 0.000000000000000000, 0.000000000000000000 ) ) ;
#3973=ORIENTED_EDGE ( 'NONE', *, *, #863, .T. ) ;
#3977=DIRECTION ( 'NONE',  ( 1.000000000000000000, 0.000000000000000000, -0.000000000000000000 ) ) ;
#3978=EDGE_CURVE ( 'NONE', #3949, #2553, #3174, .T. ) ;
#4005=DIRECTION ( 'NONE',  ( -1.000000000000000000, 0.000000000000000000, 0.000000000000000000 ) ) ;
#4027=ORIENTED_EDGE ( 'NONE', *, *, #1548, .T. ) ;
#4048=ORIENTED_EDGE ( 'NONE', *, *, #863, .F. ) ;
#4053=CARTESIAN_POINT ( 'NONE',  ( -25.99519186311192342, -0.5000000000000000000, 19.00000000000000000 ) ) ;
#4074=EDGE_LOOP ( 'NONE', ( #1755, #1542 ) ) ;
#4086=EDGE_CURVE ( 'NONE', #3949, #3182, #1939, .T. ) ;
#4121=EDGE_LOOP ( 'NONE', ( #3784, #1398, #3643, #935 ) ) ;
#4144=ORIENTED_EDGE ( 'NONE', *, *, #3978, .F. ) ;
#4149=VECTOR ( 'NONE', #888, 1000.000000000000000 ) ;
#4152=CARTESIAN_POINT ( 'NONE',  ( 26.49999999999999645, 0.5000000000000000000, 19.00000000000000000 ) ) ;
#4159=STYLED_ITEM ( 'NONE', ( #1003 ), #3930 ) ;
#4191=LINE ( 'NONE', #517, #2778 ) ;
#4198=ORIENTED_EDGE ( 'NONE', *, *, #3794, .T. ) ;
#4201=CARTESIAN_POINT ( 'NONE',  ( 26.49999999999999645, -0.5000000000000000000, 19.50000000000000000 ) ) ;
#4229=DIRECTION ( 'NONE',  ( 0.000000000000000000, 0.000000000000000000, 1.000000000000000000 ) ) ;
#4245=LINE ( 'NONE', #1346, #1236 ) ;
#4246=FACE_OUTER_BOUND ( 'NONE', #4074, .T. ) ;
#4256=DIRECTION ( 'NONE',  ( 0.000000000000000000, -0.000000000000000000, 1.000000000000000000 ) ) ;
#4264=SURFACE_SIDE_STYLE ('',( #1736 ) ) ;
#4265=CIRCLE ( 'NONE', #1442, 26.00000000000000711 ) ;
#4278=CARTESIAN_POINT ( 'NONE',  ( -25.99519186311192342, -0.5000000000000000000, 20.00000000000000000 ) ) ;
#4302=LINE ( 'NONE', #4278, #3929 ) ;
#4309=ORIENTED_EDGE ( 'NONE', *, *, #1762, .T. ) ;
#4324=DIRECTION ( 'NONE',  ( 0.000000000000000000, 1.000000000000000000, 0.000000000000000000 ) ) ;
#4333=EDGE_LOOP ( 'NONE', ( #1626, #4646, #981, #3639, #4027, #2945, #1591, #124 ) ) ;
#4337=PLANE ( 'NONE',  #437 ) ;
#4346=CARTESIAN_POINT ( 'NONE',  ( 25.99519186311192342, 0.5000000000000000000, 19.50000000000000000 ) ) ;
#4354=DIRECTION ( 'NONE',  ( 0.000000000000000000, -1.000000000000000000, -0.000000000000000000 ) ) ;
#4361=VERTEX_POINT ( 'NONE', #612 ) ;
#4362=VECTOR ( 'NONE', #2963, 1000.000000000000000 ) ;
#4380=LINE ( 'NONE', #2536, #824 ) ;
#4405=EDGE_CURVE ( 'NONE', #1759, #3886, #1410, .T. ) ;
#4420=ORIENTED_EDGE ( 'NONE', *, *, #1647, .T. ) ;
#4425=ORIENTED_EDGE ( 'NONE', *, *, #364, .T. ) ;
#4428=CARTESIAN_POINT ( 'NONE',  ( -26.50000000000000355, 0.5000000000000000000, 19.00000000000000000 ) ) ;
#4433=ORIENTED_EDGE ( 'NONE', *, *, #3978, .T. ) ;
#4467=DIRECTION ( 'NONE',  ( 0.000000000000000000, -0.000000000000000000, 1.000000000000000000 ) ) ;
#4491=CARTESIAN_POINT ( 'NONE',  ( 26.49999999999999645, 0.5000000000000000000, 19.50000000000000000 ) ) ;
#4498=VERTEX_POINT ( 'NONE', #4053 ) ;
#4511=VERTEX_POINT ( 'NONE', #1521 ) ;
#4514=AXIS2_PLACEMENT_3D ( 'NONE', #1045, #3650, #369 ) ;
#4518=DIRECTION ( 'NONE',  ( -0.000000000000000000, -1.000000000000000000, -0.000000000000000000 ) ) ;
#4529=LINE ( 'NONE', #2736, #2501 ) ;
#4543=EDGE_LOOP ( 'NONE', ( #2326, #483, #4309, #572, #1904, #835, #3212, #2754 ) ) ;
#4568=CARTESIAN_POINT ( 'NONE',  ( -26.50000000000000355, -0.5000000000000000000, 19.50000000000000000 ) ) ;
#4572=EDGE_LOOP ( 'NONE', ( #1895, #1987, #2658, #856 ) ) ;
#4575=CARTESIAN_POINT ( 'NONE',  ( 26.49999999999999645, 0.5000000000000000000, 19.50000000000000000 ) ) ;
#4584=CARTESIAN_POINT ( 'NONE',  ( 0.000000000000000000, 0.000000000000000000, 20.00000000000000000 ) ) ;
#4588=EDGE_CURVE ( 'NONE', #2553, #3303, #2685, .T. ) ;
#4596=DIRECTION ( 'NONE',  ( -1.000000000000000000, 0.000000000000000000, 0.000000000000000000 ) ) ;
#4600=DIRECTION ( 'NONE',  ( -1.000000000000000000, 0.000000000000000000, 0.000000000000000000 ) ) ;
#4646=ORIENTED_EDGE ( 'NONE', *, *, #1249, .T. ) ;
#4656=DIRECTION ( 'NONE',  ( 0.000000000000000000, -0.000000000000000000, 1.000000000000000000 ) ) ;
#4661=AXIS2_PLACEMENT_3D ( 'NONE', #234, #3134, #2151 ) ;
#4674=FACE_OUTER_BOUND ( 'NONE', #4121, .T. ) ;
#4689=PLANE ( 'NONE',  #4661 ) ;
#4692=( GEOMETRIC_REPRESENTATION_CONTEXT ( 3 ) GLOBAL_UNCERTAINTY_ASSIGNED_CONTEXT ( ( #2662 ) ) GLOBAL_UNIT_ASSIGNED_CONTEXT ( ( #2852, #3187, #627 ) ) REPRESENTATION_CONTEXT ( 'NONE', 'WORKASPACE' ) );
#4699=CARTESIAN_POINT ( 'NONE',  ( 0.000000000000000000, 0.000000000000000000, 19.50000000000000000 ) ) ;
#4706=EDGE_CURVE ( 'NONE', #4498, #2297, #2415, .T. ) ;
#4723=COLOUR_RGB('Light Blue',0.38,0.62,0.78);
#4724=FILL_AREA_STYLE_COLOUR('',#4723);
#4725=FILL_AREA_STYLE('',(#4724));
#4726=SURFACE_STYLE_FILL_AREA(#4725);
#4727=SURFACE_SIDE_STYLE('',(#4726));
#4728=SURFACE_STYLE_USAGE(.BOTH.,#4727);
#4729=PRESENTATION_STYLE_ASSIGNMENT((#4728));
ENDSEC;
END-ISO-10303-21;
